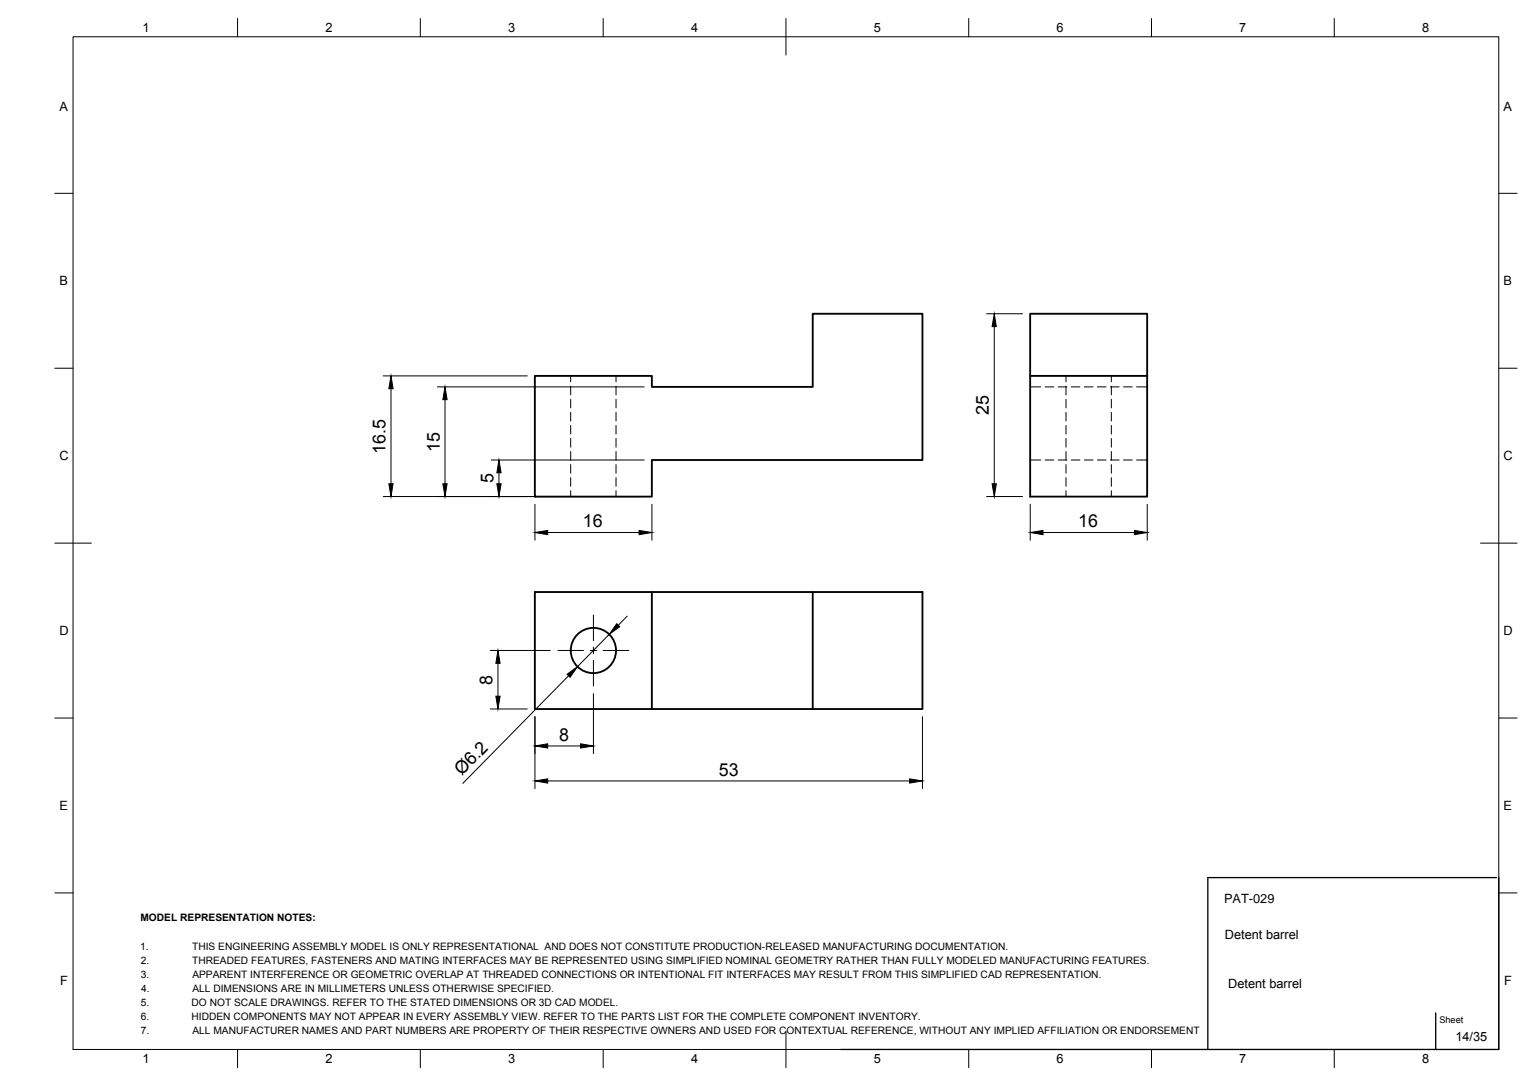
ISO-10303-21;
HEADER;
/* Generated by software containing ST-Developer
 * from STEP Tools, Inc. (www.steptools.com) 
 */

FILE_DESCRIPTION(
/* description */ ('Door-style hinge test fixture with detent'),
/* implementation_level */ '2;1');

FILE_NAME(
/* name */ 'Detent barrel.step',
/* time_stamp */ '2026-10-28T03:24:57-07:00',
/* author */ (''),
/* organization */ (''),
/* preprocessor_version */ 'ST-DEVELOPER v20.2',
/* originating_system */ 'Autodesk Translation Framework v15.17.0.0',
/* authorisation */ '');

FILE_SCHEMA (('AUTOMOTIVE_DESIGN { 1 0 10303 214 3 1 1 }'));
ENDSEC;

DATA;
#10=MECHANICAL_DESIGN_GEOMETRIC_PRESENTATION_REPRESENTATION('',(#332),#9813);
#269=SHAPE_REPRESENTATION_RELATIONSHIP('SRR','None',#9946,#300);
#300=ADVANCED_BREP_SHAPE_REPRESENTATION('',(#372),#9789);
#332=STYLED_ITEM('',(#10176),#372);
#372=MANIFOLD_SOLID_BREP('Body1',#4763);
#457=FACE_BOUND('',#1114,.T.);
#458=FACE_BOUND('',#1117,.T.);
#558=PLANE('',#5343);
#559=PLANE('',#5344);
#560=PLANE('',#5345);
#561=PLANE('',#5346);
#562=PLANE('',#5347);
#563=PLANE('',#5348);
#564=PLANE('',#5349);
#565=PLANE('',#5350);
#566=PLANE('',#5351);
#567=PLANE('',#5352);
#568=PLANE('',#5353);
#569=PLANE('',#5354);
#761=FACE_OUTER_BOUND('',#1104,.T.);
#762=FACE_OUTER_BOUND('',#1105,.T.);
#763=FACE_OUTER_BOUND('',#1106,.T.);
#764=FACE_OUTER_BOUND('',#1107,.T.);
#765=FACE_OUTER_BOUND('',#1108,.T.);
#766=FACE_OUTER_BOUND('',#1109,.T.);
#767=FACE_OUTER_BOUND('',#1110,.T.);
#768=FACE_OUTER_BOUND('',#1111,.T.);
#769=FACE_OUTER_BOUND('',#1112,.T.);
#770=FACE_OUTER_BOUND('',#1113,.T.);
#771=FACE_OUTER_BOUND('',#1115,.T.);
#772=FACE_OUTER_BOUND('',#1116,.T.);
#773=FACE_OUTER_BOUND('',#1118,.T.);
#1104=EDGE_LOOP('',(#3663,#3664,#3665,#3666));
#1105=EDGE_LOOP('',(#3667,#3668,#3669,#3670));
#1106=EDGE_LOOP('',(#3671,#3672,#3673,#3674));
#1107=EDGE_LOOP('',(#3675,#3676,#3677,#3678,#3679,#3680,#3681,#3682,#3683,
#3684));
#1108=EDGE_LOOP('',(#3685,#3686,#3687,#3688));
#1109=EDGE_LOOP('',(#3689,#3690,#3691,#3692));
#1110=EDGE_LOOP('',(#3693,#3694,#3695,#3696));
#1111=EDGE_LOOP('',(#3697,#3698,#3699,#3700));
#1112=EDGE_LOOP('',(#3701,#3702,#3703,#3704));
#1113=EDGE_LOOP('',(#3705,#3706,#3707,#3708));
#1114=EDGE_LOOP('',(#3709));
#1115=EDGE_LOOP('',(#3710,#3711,#3712,#3713));
#1116=EDGE_LOOP('',(#3714,#3715,#3716,#3717));
#1117=EDGE_LOOP('',(#3718));
#1118=EDGE_LOOP('',(#3719,#3720,#3721,#3722,#3723,#3724,#3725,#3726,#3727,
#3728));
#1470=LINE('',#7791,#1790);
#1471=LINE('',#7796,#1791);
#1472=LINE('',#7798,#1792);
#1473=LINE('',#7800,#1793);
#1474=LINE('',#7801,#1794);
#1475=LINE('',#7804,#1795);
#1476=LINE('',#7806,#1796);
#1477=LINE('',#7807,#1797);
#1478=LINE('',#7811,#1798);
#1479=LINE('',#7813,#1799);
#1480=LINE('',#7815,#1800);
#1481=LINE('',#7817,#1801);
#1482=LINE('',#7819,#1802);
#1483=LINE('',#7821,#1803);
#1484=LINE('',#7822,#1804);
#1485=LINE('',#7823,#1805);
#1486=LINE('',#7826,#1806);
#1487=LINE('',#7827,#1807);
#1488=LINE('',#7830,#1808);
#1489=LINE('',#7831,#1809);
#1490=LINE('',#7834,#1810);
#1491=LINE('',#7835,#1811);
#1492=LINE('',#7838,#1812);
#1493=LINE('',#7839,#1813);
#1494=LINE('',#7842,#1814);
#1495=LINE('',#7843,#1815);
#1496=LINE('',#7846,#1816);
#1497=LINE('',#7847,#1817);
#1498=LINE('',#7850,#1818);
#1499=LINE('',#7851,#1819);
#1500=LINE('',#7853,#1820);
#1790=VECTOR('',#6295,0.31);
#1791=VECTOR('',#6300,1.);
#1792=VECTOR('',#6301,1.);
#1793=VECTOR('',#6302,1.);
#1794=VECTOR('',#6303,1.);
#1795=VECTOR('',#6306,1.);
#1796=VECTOR('',#6307,1.);
#1797=VECTOR('',#6308,1.);
#1798=VECTOR('',#6311,1.);
#1799=VECTOR('',#6312,1.);
#1800=VECTOR('',#6313,1.);
#1801=VECTOR('',#6314,1.);
#1802=VECTOR('',#6315,1.);
#1803=VECTOR('',#6316,1.);
#1804=VECTOR('',#6317,1.);
#1805=VECTOR('',#6318,1.);
#1806=VECTOR('',#6321,1.);
#1807=VECTOR('',#6322,1.);
#1808=VECTOR('',#6325,1.);
#1809=VECTOR('',#6326,1.);
#1810=VECTOR('',#6329,1.);
#1811=VECTOR('',#6330,1.);
#1812=VECTOR('',#6333,1.);
#1813=VECTOR('',#6334,1.);
#1814=VECTOR('',#6337,1.);
#1815=VECTOR('',#6338,1.);
#1816=VECTOR('',#6341,1.);
#1817=VECTOR('',#6342,1.);
#1818=VECTOR('',#6345,1.);
#1819=VECTOR('',#6346,1.);
#1820=VECTOR('',#6349,1.);
#2066=CIRCLE('',#5341,0.31);
#2067=CIRCLE('',#5342,0.31);
#2373=VERTEX_POINT('',#7788);
#2374=VERTEX_POINT('',#7790);
#2375=VERTEX_POINT('',#7794);
#2376=VERTEX_POINT('',#7795);
#2377=VERTEX_POINT('',#7797);
#2378=VERTEX_POINT('',#7799);
#2379=VERTEX_POINT('',#7803);
#2380=VERTEX_POINT('',#7805);
#2381=VERTEX_POINT('',#7809);
#2382=VERTEX_POINT('',#7810);
#2383=VERTEX_POINT('',#7812);
#2384=VERTEX_POINT('',#7814);
#2385=VERTEX_POINT('',#7816);
#2386=VERTEX_POINT('',#7818);
#2387=VERTEX_POINT('',#7820);
#2388=VERTEX_POINT('',#7825);
#2389=VERTEX_POINT('',#7829);
#2390=VERTEX_POINT('',#7833);
#2391=VERTEX_POINT('',#7837);
#2392=VERTEX_POINT('',#7841);
#2393=VERTEX_POINT('',#7845);
#2394=VERTEX_POINT('',#7849);
#2848=EDGE_CURVE('',#2373,#2373,#2066,.T.);
#2849=EDGE_CURVE('',#2373,#2374,#1470,.T.);
#2850=EDGE_CURVE('',#2374,#2374,#2067,.T.);
#2851=EDGE_CURVE('',#2375,#2376,#1471,.T.);
#2852=EDGE_CURVE('',#2375,#2377,#1472,.T.);
#2853=EDGE_CURVE('',#2378,#2377,#1473,.T.);
#2854=EDGE_CURVE('',#2376,#2378,#1474,.T.);
#2855=EDGE_CURVE('',#2379,#2378,#1475,.T.);
#2856=EDGE_CURVE('',#2377,#2380,#1476,.T.);
#2857=EDGE_CURVE('',#2380,#2379,#1477,.T.);
#2858=EDGE_CURVE('',#2381,#2382,#1478,.T.);
#2859=EDGE_CURVE('',#2381,#2383,#1479,.T.);
#2860=EDGE_CURVE('',#2383,#2384,#1480,.T.);
#2861=EDGE_CURVE('',#2384,#2385,#1481,.T.);
#2862=EDGE_CURVE('',#2385,#2386,#1482,.T.);
#2863=EDGE_CURVE('',#2386,#2387,#1483,.T.);
#2864=EDGE_CURVE('',#2376,#2387,#1484,.T.);
#2865=EDGE_CURVE('',#2382,#2379,#1485,.T.);
#2866=EDGE_CURVE('',#2382,#2388,#1486,.T.);
#2867=EDGE_CURVE('',#2388,#2380,#1487,.T.);
#2868=EDGE_CURVE('',#2389,#2387,#1488,.T.);
#2869=EDGE_CURVE('',#2389,#2375,#1489,.T.);
#2870=EDGE_CURVE('',#2388,#2390,#1490,.T.);
#2871=EDGE_CURVE('',#2381,#2390,#1491,.T.);
#2872=EDGE_CURVE('',#2390,#2391,#1492,.T.);
#2873=EDGE_CURVE('',#2391,#2383,#1493,.T.);
#2874=EDGE_CURVE('',#2392,#2386,#1494,.T.);
#2875=EDGE_CURVE('',#2392,#2389,#1495,.T.);
#2876=EDGE_CURVE('',#2393,#2392,#1496,.T.);
#2877=EDGE_CURVE('',#2393,#2385,#1497,.T.);
#2878=EDGE_CURVE('',#2394,#2393,#1498,.T.);
#2879=EDGE_CURVE('',#2394,#2384,#1499,.T.);
#2880=EDGE_CURVE('',#2391,#2394,#1500,.T.);
#3663=ORIENTED_EDGE('',*,*,#2848,.F.);
#3664=ORIENTED_EDGE('',*,*,#2849,.T.);
#3665=ORIENTED_EDGE('',*,*,#2850,.F.);
#3666=ORIENTED_EDGE('',*,*,#2849,.F.);
#3667=ORIENTED_EDGE('',*,*,#2851,.F.);
#3668=ORIENTED_EDGE('',*,*,#2852,.T.);
#3669=ORIENTED_EDGE('',*,*,#2853,.F.);
#3670=ORIENTED_EDGE('',*,*,#2854,.F.);
#3671=ORIENTED_EDGE('',*,*,#2855,.T.);
#3672=ORIENTED_EDGE('',*,*,#2853,.T.);
#3673=ORIENTED_EDGE('',*,*,#2856,.T.);
#3674=ORIENTED_EDGE('',*,*,#2857,.T.);
#3675=ORIENTED_EDGE('',*,*,#2858,.F.);
#3676=ORIENTED_EDGE('',*,*,#2859,.T.);
#3677=ORIENTED_EDGE('',*,*,#2860,.T.);
#3678=ORIENTED_EDGE('',*,*,#2861,.T.);
#3679=ORIENTED_EDGE('',*,*,#2862,.T.);
#3680=ORIENTED_EDGE('',*,*,#2863,.T.);
#3681=ORIENTED_EDGE('',*,*,#2864,.F.);
#3682=ORIENTED_EDGE('',*,*,#2854,.T.);
#3683=ORIENTED_EDGE('',*,*,#2855,.F.);
#3684=ORIENTED_EDGE('',*,*,#2865,.F.);
#3685=ORIENTED_EDGE('',*,*,#2866,.F.);
#3686=ORIENTED_EDGE('',*,*,#2865,.T.);
#3687=ORIENTED_EDGE('',*,*,#2857,.F.);
#3688=ORIENTED_EDGE('',*,*,#2867,.F.);
#3689=ORIENTED_EDGE('',*,*,#2851,.T.);
#3690=ORIENTED_EDGE('',*,*,#2864,.T.);
#3691=ORIENTED_EDGE('',*,*,#2868,.F.);
#3692=ORIENTED_EDGE('',*,*,#2869,.T.);
#3693=ORIENTED_EDGE('',*,*,#2870,.T.);
#3694=ORIENTED_EDGE('',*,*,#2871,.F.);
#3695=ORIENTED_EDGE('',*,*,#2858,.T.);
#3696=ORIENTED_EDGE('',*,*,#2866,.T.);
#3697=ORIENTED_EDGE('',*,*,#2871,.T.);
#3698=ORIENTED_EDGE('',*,*,#2872,.T.);
#3699=ORIENTED_EDGE('',*,*,#2873,.T.);
#3700=ORIENTED_EDGE('',*,*,#2859,.F.);
#3701=ORIENTED_EDGE('',*,*,#2868,.T.);
#3702=ORIENTED_EDGE('',*,*,#2863,.F.);
#3703=ORIENTED_EDGE('',*,*,#2874,.F.);
#3704=ORIENTED_EDGE('',*,*,#2875,.T.);
#3705=ORIENTED_EDGE('',*,*,#2876,.T.);
#3706=ORIENTED_EDGE('',*,*,#2874,.T.);
#3707=ORIENTED_EDGE('',*,*,#2862,.F.);
#3708=ORIENTED_EDGE('',*,*,#2877,.F.);
#3709=ORIENTED_EDGE('',*,*,#2850,.T.);
#3710=ORIENTED_EDGE('',*,*,#2878,.T.);
#3711=ORIENTED_EDGE('',*,*,#2877,.T.);
#3712=ORIENTED_EDGE('',*,*,#2861,.F.);
#3713=ORIENTED_EDGE('',*,*,#2879,.F.);
#3714=ORIENTED_EDGE('',*,*,#2880,.T.);
#3715=ORIENTED_EDGE('',*,*,#2879,.T.);
#3716=ORIENTED_EDGE('',*,*,#2860,.F.);
#3717=ORIENTED_EDGE('',*,*,#2873,.F.);
#3718=ORIENTED_EDGE('',*,*,#2848,.T.);
#3719=ORIENTED_EDGE('',*,*,#2869,.F.);
#3720=ORIENTED_EDGE('',*,*,#2875,.F.);
#3721=ORIENTED_EDGE('',*,*,#2876,.F.);
#3722=ORIENTED_EDGE('',*,*,#2878,.F.);
#3723=ORIENTED_EDGE('',*,*,#2880,.F.);
#3724=ORIENTED_EDGE('',*,*,#2872,.F.);
#3725=ORIENTED_EDGE('',*,*,#2870,.F.);
#3726=ORIENTED_EDGE('',*,*,#2867,.T.);
#3727=ORIENTED_EDGE('',*,*,#2856,.F.);
#3728=ORIENTED_EDGE('',*,*,#2852,.F.);
#4421=CYLINDRICAL_SURFACE('',#5340,0.31);
#4566=ADVANCED_FACE('',(#761),#4421,.F.);
#4567=ADVANCED_FACE('',(#762),#558,.T.);
#4568=ADVANCED_FACE('',(#763),#559,.T.);
#4569=ADVANCED_FACE('',(#764),#560,.T.);
#4570=ADVANCED_FACE('',(#765),#561,.T.);
#4571=ADVANCED_FACE('',(#766),#562,.T.);
#4572=ADVANCED_FACE('',(#767),#563,.F.);
#4573=ADVANCED_FACE('',(#768),#564,.T.);
#4574=ADVANCED_FACE('',(#769),#565,.T.);
#4575=ADVANCED_FACE('',(#770,#457),#566,.T.);
#4576=ADVANCED_FACE('',(#771),#567,.T.);
#4577=ADVANCED_FACE('',(#772,#458),#568,.T.);
#4578=ADVANCED_FACE('',(#773),#569,.F.);
#4763=CLOSED_SHELL('',(#4566,#4567,#4568,#4569,#4570,#4571,#4572,#4573,
#4574,#4575,#4576,#4577,#4578));
#5339=AXIS2_PLACEMENT_3D('',#7786,#6289,#6290);
#5340=AXIS2_PLACEMENT_3D('',#7787,#6291,#6292);
#5341=AXIS2_PLACEMENT_3D('',#7789,#6293,#6294);
#5342=AXIS2_PLACEMENT_3D('',#7792,#6296,#6297);
#5343=AXIS2_PLACEMENT_3D('',#7793,#6298,#6299);
#5344=AXIS2_PLACEMENT_3D('',#7802,#6304,#6305);
#5345=AXIS2_PLACEMENT_3D('',#7808,#6309,#6310);
#5346=AXIS2_PLACEMENT_3D('',#7824,#6319,#6320);
#5347=AXIS2_PLACEMENT_3D('',#7828,#6323,#6324);
#5348=AXIS2_PLACEMENT_3D('',#7832,#6327,#6328);
#5349=AXIS2_PLACEMENT_3D('',#7836,#6331,#6332);
#5350=AXIS2_PLACEMENT_3D('',#7840,#6335,#6336);
#5351=AXIS2_PLACEMENT_3D('',#7844,#6339,#6340);
#5352=AXIS2_PLACEMENT_3D('',#7848,#6343,#6344);
#5353=AXIS2_PLACEMENT_3D('',#7852,#6347,#6348);
#5354=AXIS2_PLACEMENT_3D('',#7854,#6350,#6351);
#6289=DIRECTION('axis',(0.,0.,1.));
#6290=DIRECTION('refdir',(1.,0.,0.));
#6291=DIRECTION('center_axis',(0.,1.,0.));
#6292=DIRECTION('ref_axis',(1.,0.,0.));
#6293=DIRECTION('center_axis',(0.,1.,0.));
#6294=DIRECTION('ref_axis',(1.,0.,0.));
#6295=DIRECTION('',(0.,1.,0.));
#6296=DIRECTION('center_axis',(0.,-1.,0.));
#6297=DIRECTION('ref_axis',(1.,0.,0.));
#6298=DIRECTION('center_axis',(1.,0.,0.));
#6299=DIRECTION('ref_axis',(0.,0.,-1.));
#6300=DIRECTION('',(0.,0.,1.));
#6301=DIRECTION('',(0.,1.,0.));
#6302=DIRECTION('',(0.,0.,-1.));
#6303=DIRECTION('',(0.,1.,0.));
#6304=DIRECTION('center_axis',(0.,1.,0.));
#6305=DIRECTION('ref_axis',(0.,0.,1.));
#6306=DIRECTION('',(1.,0.,0.));
#6307=DIRECTION('',(-1.,0.,0.));
#6308=DIRECTION('',(0.,0.,1.));
#6309=DIRECTION('center_axis',(0.,0.,1.));
#6310=DIRECTION('ref_axis',(1.,0.,0.));
#6311=DIRECTION('',(-1.,0.,0.));
#6312=DIRECTION('',(0.,-1.,0.));
#6313=DIRECTION('',(1.,0.,0.));
#6314=DIRECTION('',(0.,1.,0.));
#6315=DIRECTION('',(-1.,0.,0.));
#6316=DIRECTION('',(0.,-1.,0.));
#6317=DIRECTION('',(1.,0.,0.));
#6318=DIRECTION('',(0.,1.,0.));
#6319=DIRECTION('center_axis',(-1.,0.,0.));
#6320=DIRECTION('ref_axis',(0.,0.,1.));
#6321=DIRECTION('',(0.,0.,-1.));
#6322=DIRECTION('',(0.,1.,0.));
#6323=DIRECTION('center_axis',(0.,1.,0.));
#6324=DIRECTION('ref_axis',(0.,0.,1.));
#6325=DIRECTION('',(0.,0.,1.));
#6326=DIRECTION('',(-1.,0.,0.));
#6327=DIRECTION('center_axis',(0.,1.,0.));
#6328=DIRECTION('ref_axis',(1.,0.,0.));
#6329=DIRECTION('',(1.,0.,0.));
#6330=DIRECTION('',(0.,0.,-1.));
#6331=DIRECTION('center_axis',(-1.,0.,0.));
#6332=DIRECTION('ref_axis',(0.,-1.,0.));
#6333=DIRECTION('',(0.,-1.,0.));
#6334=DIRECTION('',(0.,0.,1.));
#6335=DIRECTION('center_axis',(-1.,0.,0.));
#6336=DIRECTION('ref_axis',(0.,-1.,0.));
#6337=DIRECTION('',(0.,0.,1.));
#6338=DIRECTION('',(0.,-1.,0.));
#6339=DIRECTION('center_axis',(0.,1.,0.));
#6340=DIRECTION('ref_axis',(-1.,0.,0.));
#6341=DIRECTION('',(-1.,0.,0.));
#6342=DIRECTION('',(0.,0.,1.));
#6343=DIRECTION('center_axis',(1.,0.,0.));
#6344=DIRECTION('ref_axis',(0.,1.,0.));
#6345=DIRECTION('',(0.,1.,0.));
#6346=DIRECTION('',(0.,0.,1.));
#6347=DIRECTION('center_axis',(0.,-1.,0.));
#6348=DIRECTION('ref_axis',(1.,0.,0.));
#6349=DIRECTION('',(1.,0.,0.));
#6350=DIRECTION('center_axis',(0.,0.,1.));
#6351=DIRECTION('ref_axis',(1.,0.,0.));
#7786=CARTESIAN_POINT('',(0.,0.,0.));
#7787=CARTESIAN_POINT('Origin',(0.,-4.1,7.2));
#7788=CARTESIAN_POINT('',(-0.31,-4.,7.2));
#7789=CARTESIAN_POINT('Origin',(0.,-4.,7.2));
#7790=CARTESIAN_POINT('',(-0.31,-2.35,7.2));
#7791=CARTESIAN_POINT('',(-0.31,-4.1,7.2));
#7792=CARTESIAN_POINT('Origin',(0.,-2.35,7.2));
#7793=CARTESIAN_POINT('Origin',(-3.,-3.5,8.));
#7794=CARTESIAN_POINT('',(-3.,-2.5,6.4));
#7795=CARTESIAN_POINT('',(-3.,-2.5,8.));
#7796=CARTESIAN_POINT('',(-3.,-2.5,7.6));
#7797=CARTESIAN_POINT('',(-3.,-1.5,6.4));
#7798=CARTESIAN_POINT('',(-3.,-3.5,6.4));
#7799=CARTESIAN_POINT('',(-3.,-1.5,8.));
#7800=CARTESIAN_POINT('',(-3.,-1.5,6.4));
#7801=CARTESIAN_POINT('',(-3.,-3.5,8.));
#7802=CARTESIAN_POINT('Origin',(-3.75,-1.5,7.2));
#7803=CARTESIAN_POINT('',(-4.5,-1.5,8.));
#7804=CARTESIAN_POINT('',(-3.,-1.5,8.));
#7805=CARTESIAN_POINT('',(-4.5,-1.5,6.4));
#7806=CARTESIAN_POINT('',(-4.5,-1.5,6.4));
#7807=CARTESIAN_POINT('',(-4.5,-1.5,8.));
#7808=CARTESIAN_POINT('Origin',(0.,-3.175,8.));
#7809=CARTESIAN_POINT('',(-0.8,-3.5,8.));
#7810=CARTESIAN_POINT('',(-4.5,-3.5,8.));
#7811=CARTESIAN_POINT('',(-0.8,-3.5,8.));
#7812=CARTESIAN_POINT('',(-0.8,-4.,8.));
#7813=CARTESIAN_POINT('',(-0.8,-2.35,8.));
#7814=CARTESIAN_POINT('',(0.8,-4.,8.));
#7815=CARTESIAN_POINT('',(-0.8,-4.,8.));
#7816=CARTESIAN_POINT('',(0.8,-2.35,8.));
#7817=CARTESIAN_POINT('',(0.8,-4.,8.));
#7818=CARTESIAN_POINT('',(-0.8,-2.35,8.));
#7819=CARTESIAN_POINT('',(0.8,-2.35,8.));
#7820=CARTESIAN_POINT('',(-0.8,-2.5,8.));
#7821=CARTESIAN_POINT('',(-0.8,-2.35,8.));
#7822=CARTESIAN_POINT('',(-0.8,-2.5,8.));
#7823=CARTESIAN_POINT('',(-4.5,-3.5,8.));
#7824=CARTESIAN_POINT('Origin',(-4.5,-3.5,6.4));
#7825=CARTESIAN_POINT('',(-4.5,-3.5,6.4));
#7826=CARTESIAN_POINT('',(-4.5,-3.5,8.));
#7827=CARTESIAN_POINT('',(-4.5,-3.5,6.4));
#7828=CARTESIAN_POINT('Origin',(-2.65,-2.5,7.2));
#7829=CARTESIAN_POINT('',(-0.8,-2.5,6.4));
#7830=CARTESIAN_POINT('',(-0.8,-2.5,6.8));
#7831=CARTESIAN_POINT('',(-4.5,-2.5,6.4));
#7832=CARTESIAN_POINT('Origin',(-2.65,-3.5,7.2));
#7833=CARTESIAN_POINT('',(-0.8,-3.5,6.4));
#7834=CARTESIAN_POINT('',(-4.5,-3.5,6.4));
#7835=CARTESIAN_POINT('',(-0.8,-3.5,6.8));
#7836=CARTESIAN_POINT('Origin',(-0.8,-2.35,6.4));
#7837=CARTESIAN_POINT('',(-0.8,-4.,6.4));
#7838=CARTESIAN_POINT('',(-0.8,-2.35,6.4));
#7839=CARTESIAN_POINT('',(-0.8,-4.,6.4));
#7840=CARTESIAN_POINT('Origin',(-0.8,-2.35,6.4));
#7841=CARTESIAN_POINT('',(-0.8,-2.35,6.4));
#7842=CARTESIAN_POINT('',(-0.8,-2.35,6.4));
#7843=CARTESIAN_POINT('',(-0.8,-2.35,6.4));
#7844=CARTESIAN_POINT('Origin',(0.8,-2.35,6.4));
#7845=CARTESIAN_POINT('',(0.8,-2.35,6.4));
#7846=CARTESIAN_POINT('',(0.8,-2.35,6.4));
#7847=CARTESIAN_POINT('',(0.8,-2.35,6.4));
#7848=CARTESIAN_POINT('Origin',(0.8,-4.,6.4));
#7849=CARTESIAN_POINT('',(0.8,-4.,6.4));
#7850=CARTESIAN_POINT('',(0.8,-4.,6.4));
#7851=CARTESIAN_POINT('',(0.8,-4.,6.4));
#7852=CARTESIAN_POINT('Origin',(-0.8,-4.,6.4));
#7853=CARTESIAN_POINT('',(-0.8,-4.,6.4));
#7854=CARTESIAN_POINT('Origin',(0.,-3.175,6.4));
#9753=UNCERTAINTY_MEASURE_WITH_UNIT(LENGTH_MEASURE(0.001),#9814,
'DISTANCE_ACCURACY_VALUE',
'Maximum model space distance between geometric entities at asserted c
onnectivities');
#9777=UNCERTAINTY_MEASURE_WITH_UNIT(LENGTH_MEASURE(0.001),#9814,
'DISTANCE_ACCURACY_VALUE',
'Maximum model space distance between geometric entities at asserted c
onnectivities');
#9789=(
GEOMETRIC_REPRESENTATION_CONTEXT(3)
GLOBAL_UNCERTAINTY_ASSIGNED_CONTEXT((#9753))
GLOBAL_UNIT_ASSIGNED_CONTEXT((#9814,#9816,#9817))
REPRESENTATION_CONTEXT('','3D')
);
#9813=(
GEOMETRIC_REPRESENTATION_CONTEXT(3)
GLOBAL_UNCERTAINTY_ASSIGNED_CONTEXT((#9777))
GLOBAL_UNIT_ASSIGNED_CONTEXT((#9814,#9816,#9817))
REPRESENTATION_CONTEXT('','3D')
);
#9814=(
LENGTH_UNIT()
NAMED_UNIT(*)
SI_UNIT(.CENTI.,.METRE.)
);
#9816=(
NAMED_UNIT(*)
PLANE_ANGLE_UNIT()
SI_UNIT($,.RADIAN.)
);
#9817=(
NAMED_UNIT(*)
SI_UNIT($,.STERADIAN.)
SOLID_ANGLE_UNIT()
);
#9829=SHAPE_DEFINITION_REPRESENTATION(#9864,#9946);
#9864=PRODUCT_DEFINITION_SHAPE('',$,#9982);
#9946=SHAPE_REPRESENTATION('',(#5339),#9789);
#9970=PRODUCT_DEFINITION_CONTEXT('part definition',#10077,'design');
#9982=PRODUCT_DEFINITION('Detent barrel','Detent barrel',#10017,#9970);
#10017=PRODUCT_DEFINITION_FORMATION('',$,#10090);
#10077=APPLICATION_CONTEXT(
'Core Data for Automotive Mechanical Design Process');
#10078=PRODUCT_CONTEXT('part definition',#10077,'mechanical');
#10090=PRODUCT('Detent barrel','Detent barrel','Detent barrel',(#10078));
#10170=COLOUR_RGB('Sky Blue',0.24,0.69,0.87);
#10171=FILL_AREA_STYLE_COLOUR('',#10170);
#10172=FILL_AREA_STYLE('',(#10171));
#10173=SURFACE_STYLE_FILL_AREA(#10172);
#10174=SURFACE_SIDE_STYLE('',(#10173));
#10175=SURFACE_STYLE_USAGE(.BOTH.,#10174);
#10176=PRESENTATION_STYLE_ASSIGNMENT((#10175));
ENDSEC;
END-ISO-10303-21;
